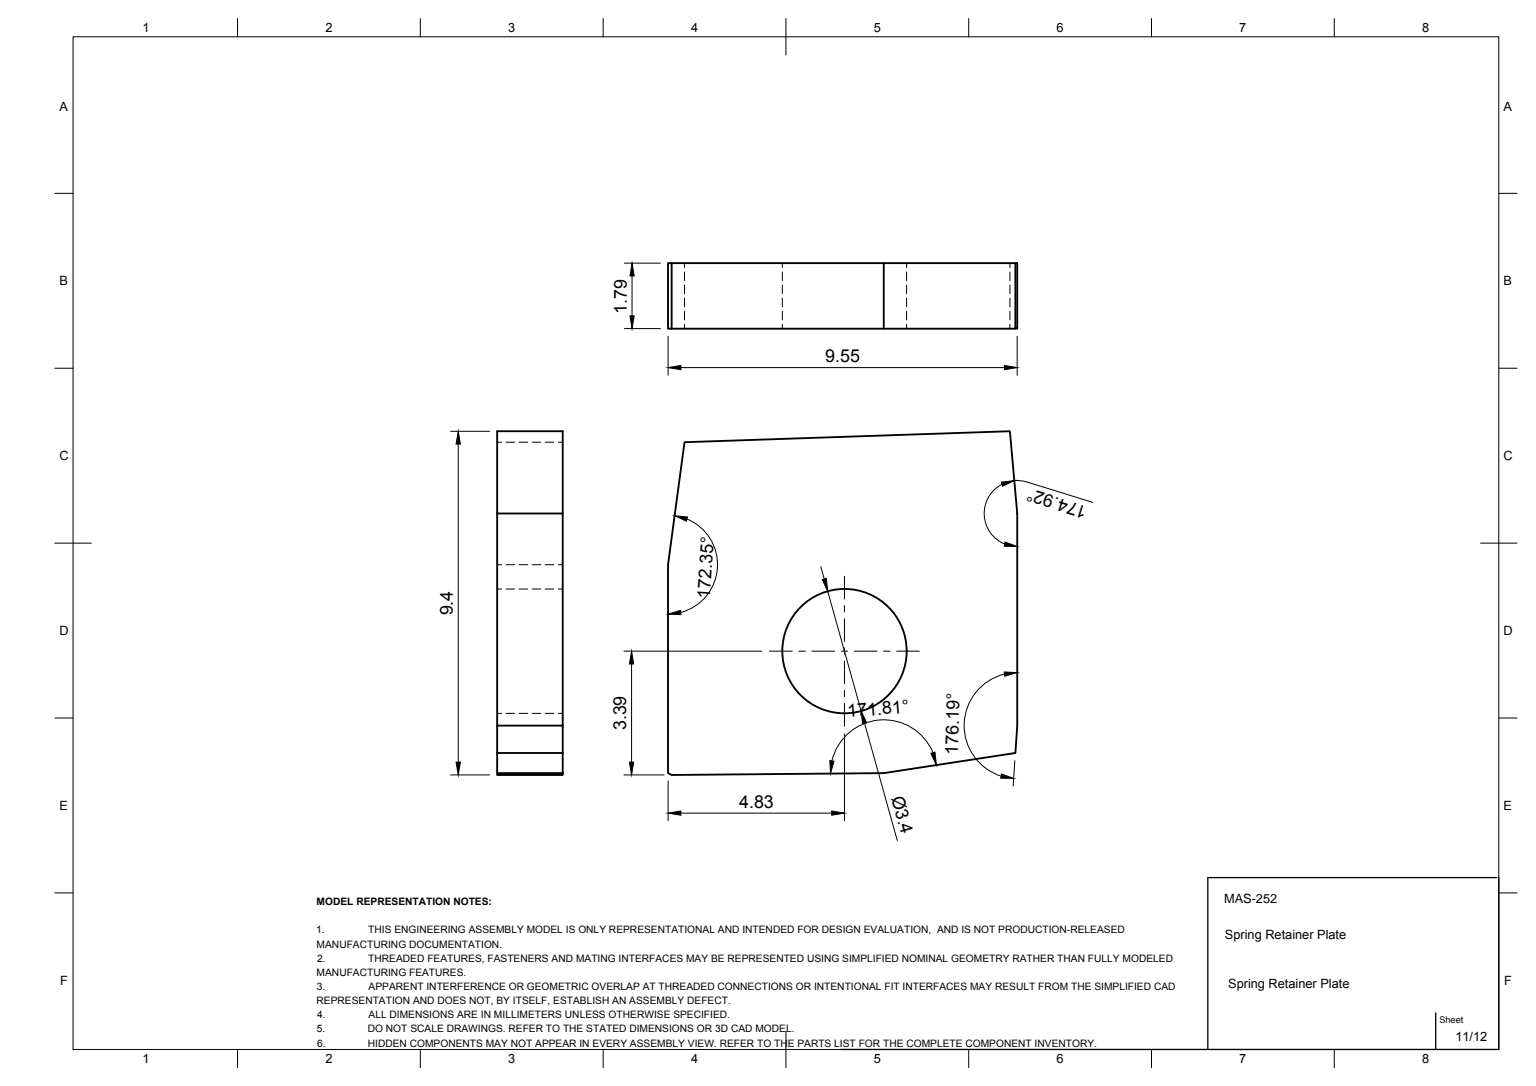
ISO-10303-21;
HEADER;
FILE_DESCRIPTION((''),'2;1');
FILE_NAME('Spring Retainer Plate.step','2026-10-06T07:01:46+05:00',(''),(''),'','','');
FILE_SCHEMA (('AUTOMOTIVE_DESIGN { 1 0 10303 214 3 1 1 }'));
ENDSEC;
DATA;
#10=MECHANICAL_DESIGN_GEOMETRIC_PRESENTATION_REPRESENTATION('',(#144),#11396);
#114=SHAPE_REPRESENTATION_RELATIONSHIP('SRR','None',#11461,#129) ;
#129=ADVANCED_BREP_SHAPE_REPRESENTATION('',(#159),#11387) ;
#144=STYLED_ITEM('',(#11545),#159) ;
#159=MANIFOLD_SOLID_BREP('Spring Retainer Plate',#5575) ;
#365=FACE_BOUND('',#1146,.T.) ;
#366=FACE_BOUND('',#1148,.T.) ;
#468=PLANE('',#6257) ;
#469=PLANE('',#6258) ;
#470=PLANE('',#6259) ;
#471=PLANE('',#6260) ;
#472=PLANE('',#6261) ;
#473=PLANE('',#6262) ;
#474=PLANE('',#6263) ;
#475=PLANE('',#6264) ;
#476=PLANE('',#6265) ;
#477=PLANE('',#6266) ;
#478=PLANE('',#6267) ;
#771=FACE_OUTER_BOUND('',#1135,.T.) ;
#772=FACE_OUTER_BOUND('',#1136,.T.) ;
#773=FACE_OUTER_BOUND('',#1137,.T.) ;
#774=FACE_OUTER_BOUND('',#1138,.T.) ;
#775=FACE_OUTER_BOUND('',#1139,.T.) ;
#776=FACE_OUTER_BOUND('',#1140,.T.) ;
#777=FACE_OUTER_BOUND('',#1141,.T.) ;
#778=FACE_OUTER_BOUND('',#1142,.T.) ;
#779=FACE_OUTER_BOUND('',#1143,.T.) ;
#780=FACE_OUTER_BOUND('',#1144,.T.) ;
#781=FACE_OUTER_BOUND('',#1145,.T.) ;
#782=FACE_OUTER_BOUND('',#1147,.T.) ;
#1135=EDGE_LOOP('',(#4766,#4767,#4768,#4769)) ;
#1136=EDGE_LOOP('',(#4770,#4771,#4772,#4773)) ;
#1137=EDGE_LOOP('',(#4774,#4775,#4776,#4777)) ;
#1138=EDGE_LOOP('',(#4778,#4779,#4780,#4781)) ;
#1139=EDGE_LOOP('',(#4782,#4783,#4784,#4785)) ;
#1140=EDGE_LOOP('',(#4786,#4787,#4788,#4789)) ;
#1141=EDGE_LOOP('',(#4790,#4791,#4792,#4793)) ;
#1142=EDGE_LOOP('',(#4794,#4795,#4796,#4797)) ;
#1143=EDGE_LOOP('',(#4798,#4799,#4800,#4801)) ;
#1144=EDGE_LOOP('',(#4802,#4803,#4804,#4805)) ;
#1145=EDGE_LOOP('',(#4806,#4807,#4808,#4809,#4810,#4811,#4812,#4813,#4814)) ;
#1146=EDGE_LOOP('',(#4815)) ;
#1147=EDGE_LOOP('',(#4816,#4817,#4818,#4819,#4820,#4821,#4822,#4823,#4824)) ;
#1148=EDGE_LOOP('',(#4825)) ;
#1506=LINE('',#10865,#1889) ;
#1507=LINE('',#10870,#1890) ;
#1508=LINE('',#10872,#1891) ;
#1509=LINE('',#10874,#1892) ;
#1510=LINE('',#10875,#1893) ;
#1511=LINE('',#10878,#1894) ;
#1512=LINE('',#10880,#1895) ;
#1513=LINE('',#10881,#1896) ;
#1514=LINE('',#10884,#1897) ;
#1515=LINE('',#10886,#1898) ;
#1516=LINE('',#10887,#1899) ;
#1517=LINE('',#10890,#1900) ;
#1518=LINE('',#10892,#1901) ;
#1519=LINE('',#10893,#1902) ;
#1520=LINE('',#10896,#1903) ;
#1521=LINE('',#10898,#1904) ;
#1522=LINE('',#10899,#1905) ;
#1523=LINE('',#10902,#1906) ;
#1524=LINE('',#10904,#1907) ;
#1525=LINE('',#10905,#1908) ;
#1526=LINE('',#10908,#1909) ;
#1527=LINE('',#10910,#1910) ;
#1528=LINE('',#10911,#1911) ;
#1529=LINE('',#10914,#1912) ;
#1530=LINE('',#10916,#1913) ;
#1531=LINE('',#10917,#1914) ;
#1532=LINE('',#10919,#1915) ;
#1533=LINE('',#10920,#1916) ;
#1889=VECTOR('',#7712,1.7) ;
#1890=VECTOR('',#7717,10.) ;
#1891=VECTOR('',#7718,10.) ;
#1892=VECTOR('',#7719,10.) ;
#1893=VECTOR('',#7720,10.) ;
#1894=VECTOR('',#7723,10.) ;
#1895=VECTOR('',#7724,10.) ;
#1896=VECTOR('',#7725,10.) ;
#1897=VECTOR('',#7728,10.) ;
#1898=VECTOR('',#7729,10.) ;
#1899=VECTOR('',#7730,10.) ;
#1900=VECTOR('',#7733,10.) ;
#1901=VECTOR('',#7734,10.) ;
#1902=VECTOR('',#7735,10.) ;
#1903=VECTOR('',#7738,10.) ;
#1904=VECTOR('',#7739,10.) ;
#1905=VECTOR('',#7740,10.) ;
#1906=VECTOR('',#7743,10.) ;
#1907=VECTOR('',#7744,10.) ;
#1908=VECTOR('',#7745,10.) ;
#1909=VECTOR('',#7748,10.) ;
#1910=VECTOR('',#7749,10.) ;
#1911=VECTOR('',#7750,10.) ;
#1912=VECTOR('',#7753,10.) ;
#1913=VECTOR('',#7754,10.) ;
#1914=VECTOR('',#7755,10.) ;
#1915=VECTOR('',#7758,10.) ;
#1916=VECTOR('',#7759,10.) ;
#2210=CIRCLE('',#6255,1.7) ;
#2211=CIRCLE('',#6256,1.7) ;
#2639=VERTEX_POINT('',#10862) ;
#2640=VERTEX_POINT('',#10864) ;
#2641=VERTEX_POINT('',#10868) ;
#2642=VERTEX_POINT('',#10869) ;
#2643=VERTEX_POINT('',#10871) ;
#2644=VERTEX_POINT('',#10873) ;
#2645=VERTEX_POINT('',#10877) ;
#2646=VERTEX_POINT('',#10879) ;
#2647=VERTEX_POINT('',#10883) ;
#2648=VERTEX_POINT('',#10885) ;
#2649=VERTEX_POINT('',#10889) ;
#2650=VERTEX_POINT('',#10891) ;
#2651=VERTEX_POINT('',#10895) ;
#2652=VERTEX_POINT('',#10897) ;
#2653=VERTEX_POINT('',#10901) ;
#2654=VERTEX_POINT('',#10903) ;
#2655=VERTEX_POINT('',#10907) ;
#2656=VERTEX_POINT('',#10909) ;
#2657=VERTEX_POINT('',#10913) ;
#2658=VERTEX_POINT('',#10915) ;
#3365=EDGE_CURVE('',#2639,#2639,#2210,.T.) ;
#3366=EDGE_CURVE('',#2639,#2640,#1506,.T.) ;
#3367=EDGE_CURVE('',#2640,#2640,#2211,.T.) ;
#3368=EDGE_CURVE('',#2641,#2642,#1507,.T.) ;
#3369=EDGE_CURVE('',#2642,#2643,#1508,.T.) ;
#3370=EDGE_CURVE('',#2644,#2643,#1509,.T.) ;
#3371=EDGE_CURVE('',#2641,#2644,#1510,.T.) ;
#3372=EDGE_CURVE('',#2645,#2641,#1511,.T.) ;
#3373=EDGE_CURVE('',#2646,#2644,#1512,.T.) ;
#3374=EDGE_CURVE('',#2645,#2646,#1513,.T.) ;
#3375=EDGE_CURVE('',#2647,#2645,#1514,.T.) ;
#3376=EDGE_CURVE('',#2648,#2646,#1515,.T.) ;
#3377=EDGE_CURVE('',#2647,#2648,#1516,.T.) ;
#3378=EDGE_CURVE('',#2649,#2647,#1517,.T.) ;
#3379=EDGE_CURVE('',#2650,#2648,#1518,.T.) ;
#3380=EDGE_CURVE('',#2649,#2650,#1519,.T.) ;
#3381=EDGE_CURVE('',#2651,#2649,#1520,.T.) ;
#3382=EDGE_CURVE('',#2652,#2650,#1521,.T.) ;
#3383=EDGE_CURVE('',#2651,#2652,#1522,.T.) ;
#3384=EDGE_CURVE('',#2653,#2651,#1523,.T.) ;
#3385=EDGE_CURVE('',#2654,#2652,#1524,.T.) ;
#3386=EDGE_CURVE('',#2653,#2654,#1525,.T.) ;
#3387=EDGE_CURVE('',#2655,#2653,#1526,.T.) ;
#3388=EDGE_CURVE('',#2656,#2654,#1527,.T.) ;
#3389=EDGE_CURVE('',#2655,#2656,#1528,.T.) ;
#3390=EDGE_CURVE('',#2657,#2655,#1529,.T.) ;
#3391=EDGE_CURVE('',#2658,#2656,#1530,.T.) ;
#3392=EDGE_CURVE('',#2657,#2658,#1531,.T.) ;
#3393=EDGE_CURVE('',#2642,#2657,#1532,.T.) ;
#3394=EDGE_CURVE('',#2643,#2658,#1533,.T.) ;
#4766=ORIENTED_EDGE('',*,*,#3365,.F.) ;
#4767=ORIENTED_EDGE('',*,*,#3366,.T.) ;
#4768=ORIENTED_EDGE('',*,*,#3367,.T.) ;
#4769=ORIENTED_EDGE('',*,*,#3366,.F.) ;
#4770=ORIENTED_EDGE('',*,*,#3368,.T.) ;
#4771=ORIENTED_EDGE('',*,*,#3369,.T.) ;
#4772=ORIENTED_EDGE('',*,*,#3370,.F.) ;
#4773=ORIENTED_EDGE('',*,*,#3371,.F.) ;
#4774=ORIENTED_EDGE('',*,*,#3372,.T.) ;
#4775=ORIENTED_EDGE('',*,*,#3371,.T.) ;
#4776=ORIENTED_EDGE('',*,*,#3373,.F.) ;
#4777=ORIENTED_EDGE('',*,*,#3374,.F.) ;
#4778=ORIENTED_EDGE('',*,*,#3375,.T.) ;
#4779=ORIENTED_EDGE('',*,*,#3374,.T.) ;
#4780=ORIENTED_EDGE('',*,*,#3376,.F.) ;
#4781=ORIENTED_EDGE('',*,*,#3377,.F.) ;
#4782=ORIENTED_EDGE('',*,*,#3378,.T.) ;
#4783=ORIENTED_EDGE('',*,*,#3377,.T.) ;
#4784=ORIENTED_EDGE('',*,*,#3379,.F.) ;
#4785=ORIENTED_EDGE('',*,*,#3380,.F.) ;
#4786=ORIENTED_EDGE('',*,*,#3381,.T.) ;
#4787=ORIENTED_EDGE('',*,*,#3380,.T.) ;
#4788=ORIENTED_EDGE('',*,*,#3382,.F.) ;
#4789=ORIENTED_EDGE('',*,*,#3383,.F.) ;
#4790=ORIENTED_EDGE('',*,*,#3384,.T.) ;
#4791=ORIENTED_EDGE('',*,*,#3383,.T.) ;
#4792=ORIENTED_EDGE('',*,*,#3385,.F.) ;
#4793=ORIENTED_EDGE('',*,*,#3386,.F.) ;
#4794=ORIENTED_EDGE('',*,*,#3387,.T.) ;
#4795=ORIENTED_EDGE('',*,*,#3386,.T.) ;
#4796=ORIENTED_EDGE('',*,*,#3388,.F.) ;
#4797=ORIENTED_EDGE('',*,*,#3389,.F.) ;
#4798=ORIENTED_EDGE('',*,*,#3390,.T.) ;
#4799=ORIENTED_EDGE('',*,*,#3389,.T.) ;
#4800=ORIENTED_EDGE('',*,*,#3391,.F.) ;
#4801=ORIENTED_EDGE('',*,*,#3392,.F.) ;
#4802=ORIENTED_EDGE('',*,*,#3393,.T.) ;
#4803=ORIENTED_EDGE('',*,*,#3392,.T.) ;
#4804=ORIENTED_EDGE('',*,*,#3394,.F.) ;
#4805=ORIENTED_EDGE('',*,*,#3369,.F.) ;
#4806=ORIENTED_EDGE('',*,*,#3394,.T.) ;
#4807=ORIENTED_EDGE('',*,*,#3391,.T.) ;
#4808=ORIENTED_EDGE('',*,*,#3388,.T.) ;
#4809=ORIENTED_EDGE('',*,*,#3385,.T.) ;
#4810=ORIENTED_EDGE('',*,*,#3382,.T.) ;
#4811=ORIENTED_EDGE('',*,*,#3379,.T.) ;
#4812=ORIENTED_EDGE('',*,*,#3376,.T.) ;
#4813=ORIENTED_EDGE('',*,*,#3373,.T.) ;
#4814=ORIENTED_EDGE('',*,*,#3370,.T.) ;
#4815=ORIENTED_EDGE('',*,*,#3365,.T.) ;
#4816=ORIENTED_EDGE('',*,*,#3393,.F.) ;
#4817=ORIENTED_EDGE('',*,*,#3368,.F.) ;
#4818=ORIENTED_EDGE('',*,*,#3372,.F.) ;
#4819=ORIENTED_EDGE('',*,*,#3375,.F.) ;
#4820=ORIENTED_EDGE('',*,*,#3378,.F.) ;
#4821=ORIENTED_EDGE('',*,*,#3381,.F.) ;
#4822=ORIENTED_EDGE('',*,*,#3384,.F.) ;
#4823=ORIENTED_EDGE('',*,*,#3387,.F.) ;
#4824=ORIENTED_EDGE('',*,*,#3390,.F.) ;
#4825=ORIENTED_EDGE('',*,*,#3367,.F.) ;
#5209=CYLINDRICAL_SURFACE('',#6254,1.7) ;
#5496=ADVANCED_FACE('',(#771),#5209,.F.) ;
#5497=ADVANCED_FACE('',(#772),#468,.T.) ;
#5498=ADVANCED_FACE('',(#773),#469,.T.) ;
#5499=ADVANCED_FACE('',(#774),#470,.T.) ;
#5500=ADVANCED_FACE('',(#775),#471,.T.) ;
#5501=ADVANCED_FACE('',(#776),#472,.T.) ;
#5502=ADVANCED_FACE('',(#777),#473,.T.) ;
#5503=ADVANCED_FACE('',(#778),#474,.T.) ;
#5504=ADVANCED_FACE('',(#779),#475,.T.) ;
#5505=ADVANCED_FACE('',(#780),#476,.T.) ;
#5506=ADVANCED_FACE('',(#781,#365),#477,.T.) ;
#5507=ADVANCED_FACE('',(#782,#366),#478,.F.) ;
#5575=CLOSED_SHELL('',(#5496,#5497,#5498,#5499,#5500,#5501,#5502,#5503,
#5504,#5505,#5506,#5507)) ;
#6253=AXIS2_PLACEMENT_3D('',#10860,#7706,#7707) ;
#6254=AXIS2_PLACEMENT_3D('',#10861,#7708,#7709) ;
#6255=AXIS2_PLACEMENT_3D('',#10863,#7710,#7711) ;
#6256=AXIS2_PLACEMENT_3D('',#10866,#7713,#7714) ;
#6257=AXIS2_PLACEMENT_3D('',#10867,#7715,#7716) ;
#6258=AXIS2_PLACEMENT_3D('',#10876,#7721,#7722) ;
#6259=AXIS2_PLACEMENT_3D('',#10882,#7726,#7727) ;
#6260=AXIS2_PLACEMENT_3D('',#10888,#7731,#7732) ;
#6261=AXIS2_PLACEMENT_3D('',#10894,#7736,#7737) ;
#6262=AXIS2_PLACEMENT_3D('',#10900,#7741,#7742) ;
#6263=AXIS2_PLACEMENT_3D('',#10906,#7746,#7747) ;
#6264=AXIS2_PLACEMENT_3D('',#10912,#7751,#7752) ;
#6265=AXIS2_PLACEMENT_3D('',#10918,#7756,#7757) ;
#6266=AXIS2_PLACEMENT_3D('',#10921,#7760,#7761) ;
#6267=AXIS2_PLACEMENT_3D('',#10922,#7762,#7763) ;
#7706=DIRECTION('axis',(0.,0.,1.)) ;
#7707=DIRECTION('refdir',(1.,0.,0.)) ;
#7708=DIRECTION('center_axis',(0.,0.,1.)) ;
#7709=DIRECTION('ref_axis',(1.,0.,0.)) ;
#7710=DIRECTION('center_axis',(0.,0.,-1.)) ;
#7711=DIRECTION('ref_axis',(1.,0.,0.)) ;
#7712=DIRECTION('',(0.,0.,-1.)) ;
#7713=DIRECTION('center_axis',(0.,0.,-1.)) ;
#7714=DIRECTION('ref_axis',(1.,0.,0.)) ;
#7715=DIRECTION('center_axis',(0.0336887316936593,0.999432373578559,0.)) ;
#7716=DIRECTION('ref_axis',(-0.999432373578559,0.0336887316936593,0.)) ;
#7717=DIRECTION('',(-0.999432373578559,0.0336887316936593,0.)) ;
#7718=DIRECTION('',(0.,0.,1.)) ;
#7719=DIRECTION('',(-0.999432373578559,0.0336887316936593,0.)) ;
#7720=DIRECTION('',(0.,0.,1.)) ;
#7721=DIRECTION('center_axis',(0.991098234868642,0.133132598713698,0.)) ;
#7722=DIRECTION('ref_axis',(-0.133132598713698,0.991098234868642,0.)) ;
#7723=DIRECTION('',(-0.133132598713698,0.991098234868642,0.)) ;
#7724=DIRECTION('',(-0.133132598713698,0.991098234868642,0.)) ;
#7725=DIRECTION('',(0.,0.,1.)) ;
#7726=DIRECTION('center_axis',(1.,0.,0.)) ;
#7727=DIRECTION('ref_axis',(0.,1.,0.)) ;
#7728=DIRECTION('',(0.,1.,0.)) ;
#7729=DIRECTION('',(0.,1.,0.)) ;
#7730=DIRECTION('',(0.,0.,1.)) ;
#7731=DIRECTION('center_axis',(0.447213595499958,-0.894427190999916,0.)) ;
#7732=DIRECTION('ref_axis',(0.894427190999916,0.447213595499958,0.)) ;
#7733=DIRECTION('',(0.894427190999916,0.447213595499958,0.)) ;
#7734=DIRECTION('',(0.894427190999916,0.447213595499958,0.)) ;
#7735=DIRECTION('',(0.,0.,1.)) ;
#7736=DIRECTION('center_axis',(-0.00862036934418878,-0.999962843925898,
0.)) ;
#7737=DIRECTION('ref_axis',(0.999962843925898,-0.00862036934418878,0.)) ;
#7738=DIRECTION('',(0.999962843925898,-0.00862036934418878,0.)) ;
#7739=DIRECTION('',(0.999962843925898,-0.00862036934418878,0.)) ;
#7740=DIRECTION('',(0.,0.,1.)) ;
#7741=DIRECTION('center_axis',(-0.151025398741513,-0.988529882671721,0.)) ;
#7742=DIRECTION('ref_axis',(0.988529882671721,-0.151025398741513,0.)) ;
#7743=DIRECTION('',(0.988529882671721,-0.151025398741513,0.)) ;
#7744=DIRECTION('',(0.988529882671721,-0.151025398741513,0.)) ;
#7745=DIRECTION('',(0.,0.,1.)) ;
#7746=DIRECTION('center_axis',(-0.997785157856609,-0.0665190105237732,0.)) ;
#7747=DIRECTION('ref_axis',(0.0665190105237732,-0.997785157856609,0.)) ;
#7748=DIRECTION('',(0.0665190105237732,-0.997785157856609,0.)) ;
#7749=DIRECTION('',(0.0665190105237732,-0.997785157856609,0.)) ;
#7750=DIRECTION('',(0.,0.,1.)) ;
#7751=DIRECTION('center_axis',(-1.,0.,0.)) ;
#7752=DIRECTION('ref_axis',(0.,-1.,0.)) ;
#7753=DIRECTION('',(0.,-1.,0.)) ;
#7754=DIRECTION('',(0.,-1.,0.)) ;
#7755=DIRECTION('',(0.,0.,1.)) ;
#7756=DIRECTION('center_axis',(-0.996072640692687,0.0885397902837945,0.)) ;
#7757=DIRECTION('ref_axis',(-0.0885397902837945,-0.996072640692687,0.)) ;
#7758=DIRECTION('',(-0.0885397902837945,-0.996072640692687,0.)) ;
#7759=DIRECTION('',(-0.0885397902837945,-0.996072640692687,0.)) ;
#7760=DIRECTION('center_axis',(0.,0.,1.)) ;
#7761=DIRECTION('ref_axis',(1.,0.,0.)) ;
#7762=DIRECTION('center_axis',(0.,0.,1.)) ;
#7763=DIRECTION('ref_axis',(1.,0.,0.)) ;
#10860=CARTESIAN_POINT('',(0.,0.,0.)) ;
#10861=CARTESIAN_POINT('Origin',(0.475,7.535,12.71)) ;
#10862=CARTESIAN_POINT('',(-1.225,7.535,14.5)) ;
#10863=CARTESIAN_POINT('Origin',(0.475,7.535,14.5)) ;
#10864=CARTESIAN_POINT('',(-1.225,7.535,12.71)) ;
#10865=CARTESIAN_POINT('',(-1.225,7.535,12.71)) ;
#10866=CARTESIAN_POINT('Origin',(0.475,7.535,12.71)) ;
#10867=CARTESIAN_POINT('Origin',(4.85,13.25,12.71)) ;
#10868=CARTESIAN_POINT('',(4.85,13.25,12.71)) ;
#10869=CARTESIAN_POINT('',(-4.05,13.55,12.71)) ;
#10870=CARTESIAN_POINT('',(4.85,13.25,12.71)) ;
#10871=CARTESIAN_POINT('',(-4.05,13.55,14.5)) ;
#10872=CARTESIAN_POINT('',(-4.05,13.55,12.71)) ;
#10873=CARTESIAN_POINT('',(4.85,13.25,14.5)) ;
#10874=CARTESIAN_POINT('',(4.85,13.25,14.5)) ;
#10875=CARTESIAN_POINT('',(4.85,13.25,12.71)) ;
#10876=CARTESIAN_POINT('Origin',(5.3,9.9,12.71)) ;
#10877=CARTESIAN_POINT('',(5.3,9.9,12.71)) ;
#10878=CARTESIAN_POINT('',(5.3,9.9,12.71)) ;
#10879=CARTESIAN_POINT('',(5.3,9.9,14.5)) ;
#10880=CARTESIAN_POINT('',(5.3,9.9,14.5)) ;
#10881=CARTESIAN_POINT('',(5.3,9.9,12.71)) ;
#10882=CARTESIAN_POINT('Origin',(5.3,4.2,12.71)) ;
#10883=CARTESIAN_POINT('',(5.3,4.2,12.71)) ;
#10884=CARTESIAN_POINT('',(5.3,4.2,12.71)) ;
#10885=CARTESIAN_POINT('',(5.3,4.2,14.5)) ;
#10886=CARTESIAN_POINT('',(5.3,4.2,14.5)) ;
#10887=CARTESIAN_POINT('',(5.3,4.2,12.71)) ;
#10888=CARTESIAN_POINT('Origin',(5.2,4.15,12.71)) ;
#10889=CARTESIAN_POINT('',(5.2,4.15,12.71)) ;
#10890=CARTESIAN_POINT('',(5.2,4.15,12.71)) ;
#10891=CARTESIAN_POINT('',(5.2,4.15,14.5)) ;
#10892=CARTESIAN_POINT('',(5.2,4.15,14.5)) ;
#10893=CARTESIAN_POINT('',(5.2,4.15,12.71)) ;
#10894=CARTESIAN_POINT('Origin',(-0.6,4.2,12.71)) ;
#10895=CARTESIAN_POINT('',(-0.6,4.2,12.71)) ;
#10896=CARTESIAN_POINT('',(-0.6,4.2,12.71)) ;
#10897=CARTESIAN_POINT('',(-0.6,4.2,14.5)) ;
#10898=CARTESIAN_POINT('',(-0.6,4.2,14.5)) ;
#10899=CARTESIAN_POINT('',(-0.6,4.2,12.71)) ;
#10900=CARTESIAN_POINT('Origin',(-4.2,4.75,12.71)) ;
#10901=CARTESIAN_POINT('',(-4.2,4.75,12.71)) ;
#10902=CARTESIAN_POINT('',(-4.2,4.75,12.71)) ;
#10903=CARTESIAN_POINT('',(-4.2,4.75,14.5)) ;
#10904=CARTESIAN_POINT('',(-4.2,4.75,14.5)) ;
#10905=CARTESIAN_POINT('',(-4.2,4.75,12.71)) ;
#10906=CARTESIAN_POINT('Origin',(-4.25,5.5,12.71)) ;
#10907=CARTESIAN_POINT('',(-4.25,5.5,12.71)) ;
#10908=CARTESIAN_POINT('',(-4.25,5.5,12.71)) ;
#10909=CARTESIAN_POINT('',(-4.25,5.5,14.5)) ;
#10910=CARTESIAN_POINT('',(-4.25,5.5,14.5)) ;
#10911=CARTESIAN_POINT('',(-4.25,5.5,12.71)) ;
#10912=CARTESIAN_POINT('Origin',(-4.25,11.3,12.71)) ;
#10913=CARTESIAN_POINT('',(-4.25,11.3,12.71)) ;
#10914=CARTESIAN_POINT('',(-4.25,11.3,12.71)) ;
#10915=CARTESIAN_POINT('',(-4.25,11.3,14.5)) ;
#10916=CARTESIAN_POINT('',(-4.25,11.3,14.5)) ;
#10917=CARTESIAN_POINT('',(-4.25,11.3,12.71)) ;
#10918=CARTESIAN_POINT('Origin',(-4.05,13.55,12.71)) ;
#10919=CARTESIAN_POINT('',(-4.05,13.55,12.71)) ;
#10920=CARTESIAN_POINT('',(-4.05,13.55,14.5)) ;
#10921=CARTESIAN_POINT('Origin',(0.525,8.85,14.5)) ;
#10922=CARTESIAN_POINT('Origin',(0.525,8.85,12.71)) ;
#11370=UNCERTAINTY_MEASURE_WITH_UNIT(LENGTH_MEASURE(0.01),#11397,
'DISTANCE_ACCURACY_VALUE',
'Maximum model space distance between geometric entities at asserted c
onnectivities') ;
#11379=UNCERTAINTY_MEASURE_WITH_UNIT(LENGTH_MEASURE(0.01),#11397,
'DISTANCE_ACCURACY_VALUE',
'Maximum model space distance between geometric entities at asserted c
onnectivities') ;
#11387=(
GEOMETRIC_REPRESENTATION_CONTEXT(3)
GLOBAL_UNCERTAINTY_ASSIGNED_CONTEXT((#11370))
GLOBAL_UNIT_ASSIGNED_CONTEXT((#11397,#11399,#11400))
REPRESENTATION_CONTEXT('','3D')
) ;
#11396=(
GEOMETRIC_REPRESENTATION_CONTEXT(3)
GLOBAL_UNCERTAINTY_ASSIGNED_CONTEXT((#11379))
GLOBAL_UNIT_ASSIGNED_CONTEXT((#11397,#11399,#11400))
REPRESENTATION_CONTEXT('','3D')
) ;
#11397=(
LENGTH_UNIT()
NAMED_UNIT(*)
SI_UNIT(.MILLI.,.METRE.)
) ;
#11399=(
NAMED_UNIT(*)
PLANE_ANGLE_UNIT()
SI_UNIT($,.RADIAN.)
) ;
#11400=(
NAMED_UNIT(*)
SI_UNIT($,.STERADIAN.)
SOLID_ANGLE_UNIT()
) ;
#11408=SHAPE_DEFINITION_REPRESENTATION(#11424,#11461) ;
#11424=PRODUCT_DEFINITION_SHAPE('',$,#11478) ;
#11461=SHAPE_REPRESENTATION('',(#6253),#11387) ;
#11470=PRODUCT_DEFINITION_CONTEXT('part definition',#11520,'design') ;
#11478=PRODUCT_DEFINITION('Spring Retainer Plate',
'Spring Retainer Plate',#11494,#11470) ;
#11494=PRODUCT_DEFINITION_FORMATION('',$,#11529) ;
#11520=APPLICATION_CONTEXT(
'Core Data for Automotive Mechanical Design Process') ;
#11521=PRODUCT_CONTEXT('part definition',#11520,'mechanical') ;
#11529=PRODUCT('Spring Retainer Plate','Spring Retainer Plate',$,(#11521)) ;
#11545=PRESENTATION_STYLE_ASSIGNMENT((#11561)) ;
#11561=SURFACE_STYLE_USAGE(.BOTH.,#11577) ;
#11577=SURFACE_SIDE_STYLE('',(#11593)) ;
#11593=SURFACE_STYLE_FILL_AREA(#11609) ;
#11609=FILL_AREA_STYLE('MAS-252 Metallic - Spring Retainer Plate',(#11625)) ;
#11625=FILL_AREA_STYLE_COLOUR(
'MAS-252 Metallic - Spring Retainer Plate',#11641) ;
#11641=COLOUR_RGB('MAS-252 Metallic - Spring Retainer Plate', 0.09019608, 0.27058824, 0.51372549) ;
ENDSEC;
END-ISO-10303-21;
